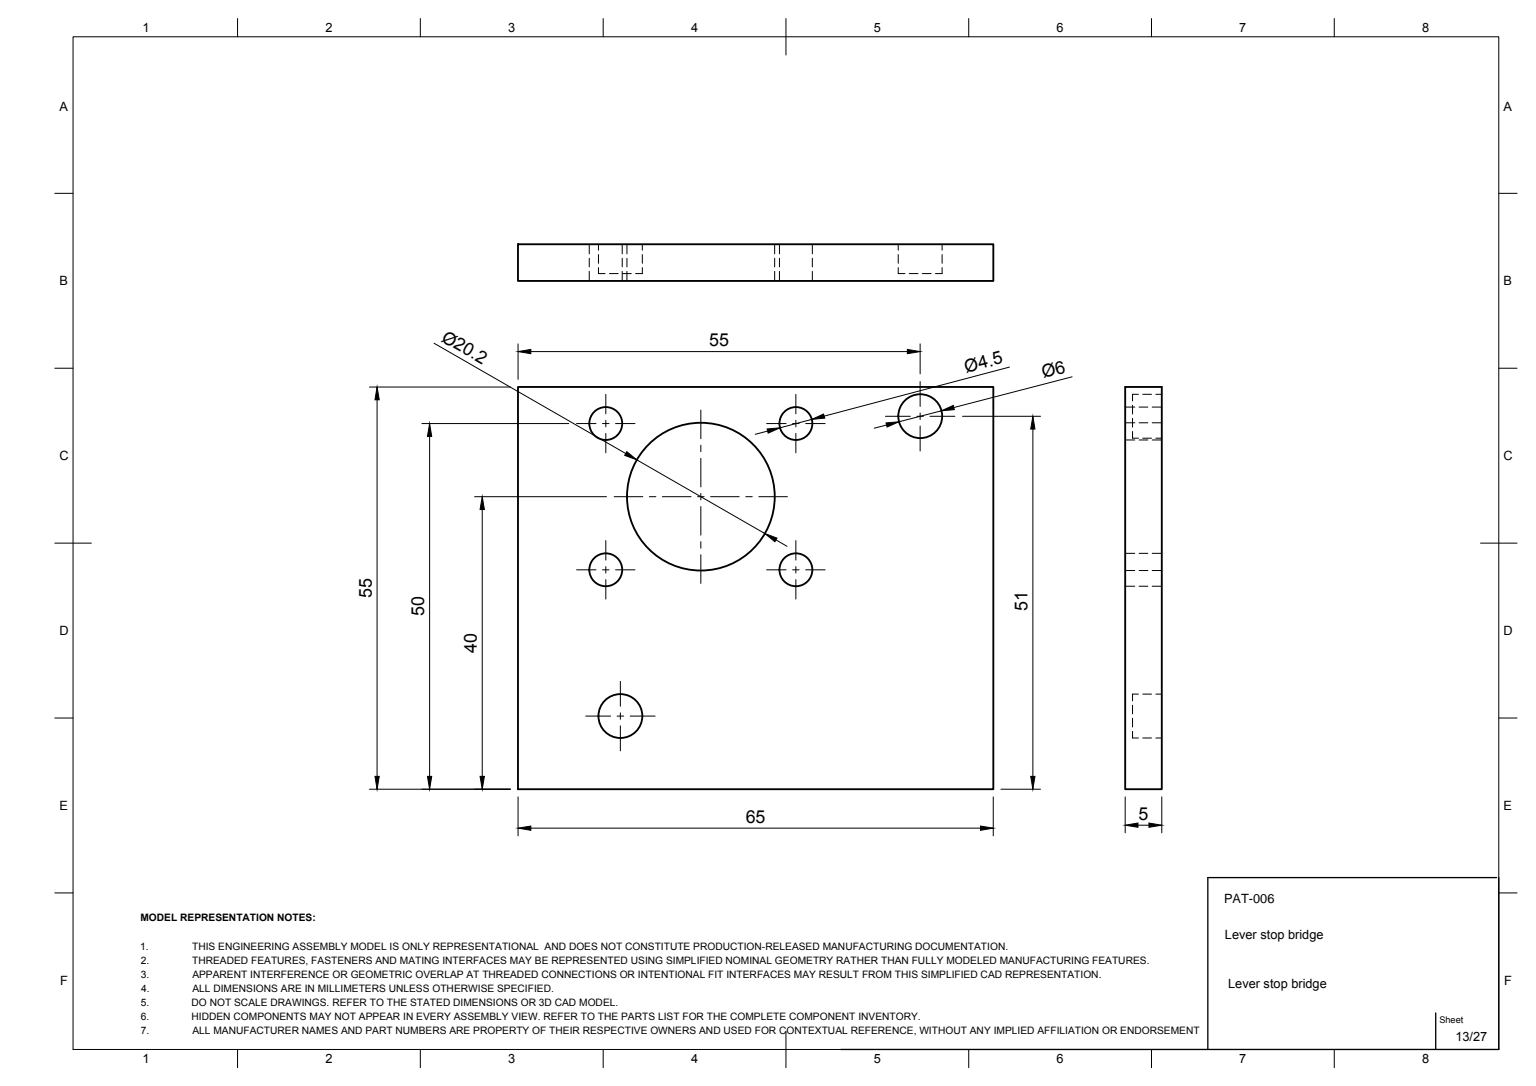
ISO-10303-21;
HEADER;
/* Generated by software containing ST-Developer
 * from STEP Tools, Inc. (www.steptools.com) 
 */

FILE_DESCRIPTION(
/* description */ ('Ball-type isolation valve (generic)'),
/* implementation_level */ '2;1');

FILE_NAME(
/* name */ 'Lever stop bridge.step',
/* time_stamp */ '2026-10-27T10:53:05-07:00',
/* author */ (''),
/* organization */ (''),
/* preprocessor_version */ 'ST-DEVELOPER v20.2',
/* originating_system */ 'Autodesk Translation Framework v15.17.0.0',
/* authorisation */ '');

FILE_SCHEMA (('AUTOMOTIVE_DESIGN { 1 0 10303 214 3 1 1 }'));
ENDSEC;

DATA;
#10=MECHANICAL_DESIGN_GEOMETRIC_PRESENTATION_REPRESENTATION('',(#285),#7425);
#233=SHAPE_REPRESENTATION_RELATIONSHIP('SRR','None',#7543,#259);
#259=ADVANCED_BREP_SHAPE_REPRESENTATION('',(#311),#7406);
#285=STYLED_ITEM('',(#7730),#311);
#311=MANIFOLD_SOLID_BREP('Body1',#4090);
#379=FACE_BOUND('',#971,.T.);
#380=FACE_BOUND('',#972,.T.);
#381=FACE_BOUND('',#973,.T.);
#382=FACE_BOUND('',#974,.T.);
#383=FACE_BOUND('',#975,.T.);
#384=FACE_BOUND('',#976,.T.);
#385=FACE_BOUND('',#977,.T.);
#386=FACE_BOUND('',#979,.T.);
#387=FACE_BOUND('',#980,.T.);
#388=FACE_BOUND('',#981,.T.);
#389=FACE_BOUND('',#982,.T.);
#390=FACE_BOUND('',#983,.T.);
#462=PLANE('',#4569);
#463=PLANE('',#4573);
#464=PLANE('',#4589);
#465=PLANE('',#4590);
#466=PLANE('',#4591);
#467=PLANE('',#4592);
#468=PLANE('',#4593);
#469=PLANE('',#4594);
#660=FACE_OUTER_BOUND('',#957,.T.);
#661=FACE_OUTER_BOUND('',#958,.T.);
#662=FACE_OUTER_BOUND('',#959,.T.);
#663=FACE_OUTER_BOUND('',#960,.T.);
#664=FACE_OUTER_BOUND('',#961,.T.);
#665=FACE_OUTER_BOUND('',#962,.T.);
#666=FACE_OUTER_BOUND('',#963,.T.);
#667=FACE_OUTER_BOUND('',#964,.T.);
#668=FACE_OUTER_BOUND('',#965,.T.);
#669=FACE_OUTER_BOUND('',#966,.T.);
#670=FACE_OUTER_BOUND('',#967,.T.);
#671=FACE_OUTER_BOUND('',#968,.T.);
#672=FACE_OUTER_BOUND('',#969,.T.);
#673=FACE_OUTER_BOUND('',#970,.T.);
#674=FACE_OUTER_BOUND('',#978,.T.);
#957=EDGE_LOOP('',(#3111,#3112,#3113,#3114));
#958=EDGE_LOOP('',(#3115));
#959=EDGE_LOOP('',(#3116,#3117,#3118,#3119));
#960=EDGE_LOOP('',(#3120));
#961=EDGE_LOOP('',(#3121,#3122,#3123,#3124));
#962=EDGE_LOOP('',(#3125,#3126,#3127,#3128));
#963=EDGE_LOOP('',(#3129,#3130,#3131,#3132));
#964=EDGE_LOOP('',(#3133,#3134,#3135,#3136));
#965=EDGE_LOOP('',(#3137,#3138,#3139,#3140));
#966=EDGE_LOOP('',(#3141,#3142,#3143,#3144));
#967=EDGE_LOOP('',(#3145,#3146,#3147,#3148));
#968=EDGE_LOOP('',(#3149,#3150,#3151,#3152));
#969=EDGE_LOOP('',(#3153,#3154,#3155,#3156));
#970=EDGE_LOOP('',(#3157,#3158,#3159,#3160));
#971=EDGE_LOOP('',(#3161));
#972=EDGE_LOOP('',(#3162));
#973=EDGE_LOOP('',(#3163));
#974=EDGE_LOOP('',(#3164));
#975=EDGE_LOOP('',(#3165));
#976=EDGE_LOOP('',(#3166));
#977=EDGE_LOOP('',(#3167));
#978=EDGE_LOOP('',(#3168,#3169,#3170,#3171));
#979=EDGE_LOOP('',(#3172));
#980=EDGE_LOOP('',(#3173));
#981=EDGE_LOOP('',(#3174));
#982=EDGE_LOOP('',(#3175));
#983=EDGE_LOOP('',(#3176));
#1257=LINE('',#6577,#1565);
#1258=LINE('',#6584,#1566);
#1259=LINE('',#6591,#1567);
#1260=LINE('',#6597,#1568);
#1261=LINE('',#6603,#1569);
#1262=LINE('',#6609,#1570);
#1263=LINE('',#6615,#1571);
#1264=LINE('',#6620,#1572);
#1265=LINE('',#6622,#1573);
#1266=LINE('',#6624,#1574);
#1267=LINE('',#6625,#1575);
#1268=LINE('',#6628,#1576);
#1269=LINE('',#6630,#1577);
#1270=LINE('',#6631,#1578);
#1271=LINE('',#6634,#1579);
#1272=LINE('',#6636,#1580);
#1273=LINE('',#6637,#1581);
#1274=LINE('',#6639,#1582);
#1275=LINE('',#6640,#1583);
#1565=VECTOR('',#5328,0.3);
#1566=VECTOR('',#5337,0.3);
#1567=VECTOR('',#5346,0.225);
#1568=VECTOR('',#5353,0.225);
#1569=VECTOR('',#5360,0.225);
#1570=VECTOR('',#5367,0.225);
#1571=VECTOR('',#5374,1.01);
#1572=VECTOR('',#5379,1.);
#1573=VECTOR('',#5380,1.);
#1574=VECTOR('',#5381,1.);
#1575=VECTOR('',#5382,1.);
#1576=VECTOR('',#5385,1.);
#1577=VECTOR('',#5386,1.);
#1578=VECTOR('',#5387,1.);
#1579=VECTOR('',#5390,1.);
#1580=VECTOR('',#5391,1.);
#1581=VECTOR('',#5392,1.);
#1582=VECTOR('',#5395,1.);
#1583=VECTOR('',#5396,1.);
#1857=CIRCLE('',#4567,0.3);
#1858=CIRCLE('',#4568,0.3);
#1859=CIRCLE('',#4571,0.3);
#1860=CIRCLE('',#4572,0.3);
#1861=CIRCLE('',#4575,0.225);
#1862=CIRCLE('',#4576,0.225);
#1863=CIRCLE('',#4578,0.225);
#1864=CIRCLE('',#4579,0.225);
#1865=CIRCLE('',#4581,0.225);
#1866=CIRCLE('',#4582,0.225);
#1867=CIRCLE('',#4584,0.225);
#1868=CIRCLE('',#4585,0.225);
#1869=CIRCLE('',#4587,1.01);
#1870=CIRCLE('',#4588,1.01);
#2069=VERTEX_POINT('',#6574);
#2070=VERTEX_POINT('',#6576);
#2071=VERTEX_POINT('',#6581);
#2072=VERTEX_POINT('',#6583);
#2073=VERTEX_POINT('',#6588);
#2074=VERTEX_POINT('',#6590);
#2075=VERTEX_POINT('',#6594);
#2076=VERTEX_POINT('',#6596);
#2077=VERTEX_POINT('',#6600);
#2078=VERTEX_POINT('',#6602);
#2079=VERTEX_POINT('',#6606);
#2080=VERTEX_POINT('',#6608);
#2081=VERTEX_POINT('',#6612);
#2082=VERTEX_POINT('',#6614);
#2083=VERTEX_POINT('',#6618);
#2084=VERTEX_POINT('',#6619);
#2085=VERTEX_POINT('',#6621);
#2086=VERTEX_POINT('',#6623);
#2087=VERTEX_POINT('',#6627);
#2088=VERTEX_POINT('',#6629);
#2089=VERTEX_POINT('',#6633);
#2090=VERTEX_POINT('',#6635);
#2448=EDGE_CURVE('',#2069,#2069,#1857,.T.);
#2449=EDGE_CURVE('',#2069,#2070,#1257,.T.);
#2450=EDGE_CURVE('',#2070,#2070,#1858,.T.);
#2451=EDGE_CURVE('',#2071,#2071,#1859,.T.);
#2452=EDGE_CURVE('',#2071,#2072,#1258,.T.);
#2453=EDGE_CURVE('',#2072,#2072,#1860,.T.);
#2454=EDGE_CURVE('',#2073,#2073,#1861,.T.);
#2455=EDGE_CURVE('',#2073,#2074,#1259,.T.);
#2456=EDGE_CURVE('',#2074,#2074,#1862,.T.);
#2457=EDGE_CURVE('',#2075,#2075,#1863,.T.);
#2458=EDGE_CURVE('',#2075,#2076,#1260,.T.);
#2459=EDGE_CURVE('',#2076,#2076,#1864,.T.);
#2460=EDGE_CURVE('',#2077,#2077,#1865,.T.);
#2461=EDGE_CURVE('',#2077,#2078,#1261,.T.);
#2462=EDGE_CURVE('',#2078,#2078,#1866,.T.);
#2463=EDGE_CURVE('',#2079,#2079,#1867,.T.);
#2464=EDGE_CURVE('',#2079,#2080,#1262,.T.);
#2465=EDGE_CURVE('',#2080,#2080,#1868,.T.);
#2466=EDGE_CURVE('',#2081,#2081,#1869,.T.);
#2467=EDGE_CURVE('',#2081,#2082,#1263,.T.);
#2468=EDGE_CURVE('',#2082,#2082,#1870,.T.);
#2469=EDGE_CURVE('',#2083,#2084,#1264,.T.);
#2470=EDGE_CURVE('',#2084,#2085,#1265,.T.);
#2471=EDGE_CURVE('',#2086,#2085,#1266,.T.);
#2472=EDGE_CURVE('',#2083,#2086,#1267,.T.);
#2473=EDGE_CURVE('',#2087,#2083,#1268,.T.);
#2474=EDGE_CURVE('',#2088,#2086,#1269,.T.);
#2475=EDGE_CURVE('',#2087,#2088,#1270,.T.);
#2476=EDGE_CURVE('',#2089,#2087,#1271,.T.);
#2477=EDGE_CURVE('',#2090,#2088,#1272,.T.);
#2478=EDGE_CURVE('',#2089,#2090,#1273,.T.);
#2479=EDGE_CURVE('',#2084,#2089,#1274,.T.);
#2480=EDGE_CURVE('',#2085,#2090,#1275,.T.);
#3111=ORIENTED_EDGE('',*,*,#2448,.F.);
#3112=ORIENTED_EDGE('',*,*,#2449,.T.);
#3113=ORIENTED_EDGE('',*,*,#2450,.F.);
#3114=ORIENTED_EDGE('',*,*,#2449,.F.);
#3115=ORIENTED_EDGE('',*,*,#2448,.T.);
#3116=ORIENTED_EDGE('',*,*,#2451,.F.);
#3117=ORIENTED_EDGE('',*,*,#2452,.T.);
#3118=ORIENTED_EDGE('',*,*,#2453,.F.);
#3119=ORIENTED_EDGE('',*,*,#2452,.F.);
#3120=ORIENTED_EDGE('',*,*,#2451,.T.);
#3121=ORIENTED_EDGE('',*,*,#2454,.F.);
#3122=ORIENTED_EDGE('',*,*,#2455,.T.);
#3123=ORIENTED_EDGE('',*,*,#2456,.F.);
#3124=ORIENTED_EDGE('',*,*,#2455,.F.);
#3125=ORIENTED_EDGE('',*,*,#2457,.F.);
#3126=ORIENTED_EDGE('',*,*,#2458,.T.);
#3127=ORIENTED_EDGE('',*,*,#2459,.F.);
#3128=ORIENTED_EDGE('',*,*,#2458,.F.);
#3129=ORIENTED_EDGE('',*,*,#2460,.F.);
#3130=ORIENTED_EDGE('',*,*,#2461,.T.);
#3131=ORIENTED_EDGE('',*,*,#2462,.F.);
#3132=ORIENTED_EDGE('',*,*,#2461,.F.);
#3133=ORIENTED_EDGE('',*,*,#2463,.F.);
#3134=ORIENTED_EDGE('',*,*,#2464,.T.);
#3135=ORIENTED_EDGE('',*,*,#2465,.F.);
#3136=ORIENTED_EDGE('',*,*,#2464,.F.);
#3137=ORIENTED_EDGE('',*,*,#2466,.F.);
#3138=ORIENTED_EDGE('',*,*,#2467,.T.);
#3139=ORIENTED_EDGE('',*,*,#2468,.F.);
#3140=ORIENTED_EDGE('',*,*,#2467,.F.);
#3141=ORIENTED_EDGE('',*,*,#2469,.T.);
#3142=ORIENTED_EDGE('',*,*,#2470,.T.);
#3143=ORIENTED_EDGE('',*,*,#2471,.F.);
#3144=ORIENTED_EDGE('',*,*,#2472,.F.);
#3145=ORIENTED_EDGE('',*,*,#2473,.T.);
#3146=ORIENTED_EDGE('',*,*,#2472,.T.);
#3147=ORIENTED_EDGE('',*,*,#2474,.F.);
#3148=ORIENTED_EDGE('',*,*,#2475,.F.);
#3149=ORIENTED_EDGE('',*,*,#2476,.T.);
#3150=ORIENTED_EDGE('',*,*,#2475,.T.);
#3151=ORIENTED_EDGE('',*,*,#2477,.F.);
#3152=ORIENTED_EDGE('',*,*,#2478,.F.);
#3153=ORIENTED_EDGE('',*,*,#2479,.T.);
#3154=ORIENTED_EDGE('',*,*,#2478,.T.);
#3155=ORIENTED_EDGE('',*,*,#2480,.F.);
#3156=ORIENTED_EDGE('',*,*,#2470,.F.);
#3157=ORIENTED_EDGE('',*,*,#2480,.T.);
#3158=ORIENTED_EDGE('',*,*,#2477,.T.);
#3159=ORIENTED_EDGE('',*,*,#2474,.T.);
#3160=ORIENTED_EDGE('',*,*,#2471,.T.);
#3161=ORIENTED_EDGE('',*,*,#2450,.T.);
#3162=ORIENTED_EDGE('',*,*,#2453,.T.);
#3163=ORIENTED_EDGE('',*,*,#2468,.T.);
#3164=ORIENTED_EDGE('',*,*,#2465,.T.);
#3165=ORIENTED_EDGE('',*,*,#2462,.T.);
#3166=ORIENTED_EDGE('',*,*,#2459,.T.);
#3167=ORIENTED_EDGE('',*,*,#2456,.T.);
#3168=ORIENTED_EDGE('',*,*,#2479,.F.);
#3169=ORIENTED_EDGE('',*,*,#2469,.F.);
#3170=ORIENTED_EDGE('',*,*,#2473,.F.);
#3171=ORIENTED_EDGE('',*,*,#2476,.F.);
#3172=ORIENTED_EDGE('',*,*,#2466,.T.);
#3173=ORIENTED_EDGE('',*,*,#2463,.T.);
#3174=ORIENTED_EDGE('',*,*,#2460,.T.);
#3175=ORIENTED_EDGE('',*,*,#2457,.T.);
#3176=ORIENTED_EDGE('',*,*,#2454,.T.);
#3798=CYLINDRICAL_SURFACE('',#4566,0.3);
#3799=CYLINDRICAL_SURFACE('',#4570,0.3);
#3800=CYLINDRICAL_SURFACE('',#4574,0.225);
#3801=CYLINDRICAL_SURFACE('',#4577,0.225);
#3802=CYLINDRICAL_SURFACE('',#4580,0.225);
#3803=CYLINDRICAL_SURFACE('',#4583,0.225);
#3804=CYLINDRICAL_SURFACE('',#4586,1.01);
#3914=ADVANCED_FACE('',(#660),#3798,.F.);
#3915=ADVANCED_FACE('',(#661),#462,.T.);
#3916=ADVANCED_FACE('',(#662),#3799,.F.);
#3917=ADVANCED_FACE('',(#663),#463,.T.);
#3918=ADVANCED_FACE('',(#664),#3800,.F.);
#3919=ADVANCED_FACE('',(#665),#3801,.F.);
#3920=ADVANCED_FACE('',(#666),#3802,.F.);
#3921=ADVANCED_FACE('',(#667),#3803,.F.);
#3922=ADVANCED_FACE('',(#668),#3804,.F.);
#3923=ADVANCED_FACE('',(#669),#464,.T.);
#3924=ADVANCED_FACE('',(#670),#465,.T.);
#3925=ADVANCED_FACE('',(#671),#466,.T.);
#3926=ADVANCED_FACE('',(#672),#467,.T.);
#3927=ADVANCED_FACE('',(#673,#379,#380,#381,#382,#383,#384,#385),#468,.T.);
#3928=ADVANCED_FACE('',(#674,#386,#387,#388,#389,#390),#469,.F.);
#4090=CLOSED_SHELL('',(#3914,#3915,#3916,#3917,#3918,#3919,#3920,#3921,
#3922,#3923,#3924,#3925,#3926,#3927,#3928));
#4565=AXIS2_PLACEMENT_3D('',#6572,#5322,#5323);
#4566=AXIS2_PLACEMENT_3D('',#6573,#5324,#5325);
#4567=AXIS2_PLACEMENT_3D('',#6575,#5326,#5327);
#4568=AXIS2_PLACEMENT_3D('',#6578,#5329,#5330);
#4569=AXIS2_PLACEMENT_3D('',#6579,#5331,#5332);
#4570=AXIS2_PLACEMENT_3D('',#6580,#5333,#5334);
#4571=AXIS2_PLACEMENT_3D('',#6582,#5335,#5336);
#4572=AXIS2_PLACEMENT_3D('',#6585,#5338,#5339);
#4573=AXIS2_PLACEMENT_3D('',#6586,#5340,#5341);
#4574=AXIS2_PLACEMENT_3D('',#6587,#5342,#5343);
#4575=AXIS2_PLACEMENT_3D('',#6589,#5344,#5345);
#4576=AXIS2_PLACEMENT_3D('',#6592,#5347,#5348);
#4577=AXIS2_PLACEMENT_3D('',#6593,#5349,#5350);
#4578=AXIS2_PLACEMENT_3D('',#6595,#5351,#5352);
#4579=AXIS2_PLACEMENT_3D('',#6598,#5354,#5355);
#4580=AXIS2_PLACEMENT_3D('',#6599,#5356,#5357);
#4581=AXIS2_PLACEMENT_3D('',#6601,#5358,#5359);
#4582=AXIS2_PLACEMENT_3D('',#6604,#5361,#5362);
#4583=AXIS2_PLACEMENT_3D('',#6605,#5363,#5364);
#4584=AXIS2_PLACEMENT_3D('',#6607,#5365,#5366);
#4585=AXIS2_PLACEMENT_3D('',#6610,#5368,#5369);
#4586=AXIS2_PLACEMENT_3D('',#6611,#5370,#5371);
#4587=AXIS2_PLACEMENT_3D('',#6613,#5372,#5373);
#4588=AXIS2_PLACEMENT_3D('',#6616,#5375,#5376);
#4589=AXIS2_PLACEMENT_3D('',#6617,#5377,#5378);
#4590=AXIS2_PLACEMENT_3D('',#6626,#5383,#5384);
#4591=AXIS2_PLACEMENT_3D('',#6632,#5388,#5389);
#4592=AXIS2_PLACEMENT_3D('',#6638,#5393,#5394);
#4593=AXIS2_PLACEMENT_3D('',#6641,#5397,#5398);
#4594=AXIS2_PLACEMENT_3D('',#6642,#5399,#5400);
#5322=DIRECTION('axis',(0.,0.,1.));
#5323=DIRECTION('refdir',(1.,0.,0.));
#5324=DIRECTION('center_axis',(0.,0.,1.));
#5325=DIRECTION('ref_axis',(1.,0.,0.));
#5326=DIRECTION('center_axis',(0.,0.,1.));
#5327=DIRECTION('ref_axis',(1.,0.,0.));
#5328=DIRECTION('',(0.,0.,1.));
#5329=DIRECTION('center_axis',(0.,0.,-1.));
#5330=DIRECTION('ref_axis',(1.,0.,0.));
#5331=DIRECTION('center_axis',(0.,0.,1.));
#5332=DIRECTION('ref_axis',(1.,0.,0.));
#5333=DIRECTION('center_axis',(0.,0.,1.));
#5334=DIRECTION('ref_axis',(1.,0.,0.));
#5335=DIRECTION('center_axis',(0.,0.,1.));
#5336=DIRECTION('ref_axis',(1.,0.,0.));
#5337=DIRECTION('',(0.,0.,1.));
#5338=DIRECTION('center_axis',(0.,0.,-1.));
#5339=DIRECTION('ref_axis',(1.,0.,0.));
#5340=DIRECTION('center_axis',(0.,0.,1.));
#5341=DIRECTION('ref_axis',(1.,0.,0.));
#5342=DIRECTION('center_axis',(0.,0.,1.));
#5343=DIRECTION('ref_axis',(1.,0.,0.));
#5344=DIRECTION('center_axis',(0.,0.,1.));
#5345=DIRECTION('ref_axis',(1.,0.,0.));
#5346=DIRECTION('',(0.,0.,1.));
#5347=DIRECTION('center_axis',(0.,0.,-1.));
#5348=DIRECTION('ref_axis',(1.,0.,0.));
#5349=DIRECTION('center_axis',(0.,0.,1.));
#5350=DIRECTION('ref_axis',(1.,0.,0.));
#5351=DIRECTION('center_axis',(0.,0.,1.));
#5352=DIRECTION('ref_axis',(1.,0.,0.));
#5353=DIRECTION('',(0.,0.,1.));
#5354=DIRECTION('center_axis',(0.,0.,-1.));
#5355=DIRECTION('ref_axis',(1.,0.,0.));
#5356=DIRECTION('center_axis',(0.,0.,1.));
#5357=DIRECTION('ref_axis',(1.,0.,0.));
#5358=DIRECTION('center_axis',(0.,0.,1.));
#5359=DIRECTION('ref_axis',(1.,0.,0.));
#5360=DIRECTION('',(0.,0.,1.));
#5361=DIRECTION('center_axis',(0.,0.,-1.));
#5362=DIRECTION('ref_axis',(1.,0.,0.));
#5363=DIRECTION('center_axis',(0.,0.,1.));
#5364=DIRECTION('ref_axis',(1.,0.,0.));
#5365=DIRECTION('center_axis',(0.,0.,1.));
#5366=DIRECTION('ref_axis',(1.,0.,0.));
#5367=DIRECTION('',(0.,0.,1.));
#5368=DIRECTION('center_axis',(0.,0.,-1.));
#5369=DIRECTION('ref_axis',(1.,0.,0.));
#5370=DIRECTION('center_axis',(0.,0.,1.));
#5371=DIRECTION('ref_axis',(1.,0.,0.));
#5372=DIRECTION('center_axis',(0.,0.,1.));
#5373=DIRECTION('ref_axis',(1.,0.,0.));
#5374=DIRECTION('',(0.,0.,1.));
#5375=DIRECTION('center_axis',(0.,0.,-1.));
#5376=DIRECTION('ref_axis',(1.,0.,0.));
#5377=DIRECTION('center_axis',(0.,1.,0.));
#5378=DIRECTION('ref_axis',(-1.,0.,0.));
#5379=DIRECTION('',(-1.,0.,0.));
#5380=DIRECTION('',(0.,0.,1.));
#5381=DIRECTION('',(-1.,0.,0.));
#5382=DIRECTION('',(0.,0.,1.));
#5383=DIRECTION('center_axis',(1.,0.,0.));
#5384=DIRECTION('ref_axis',(0.,1.,0.));
#5385=DIRECTION('',(0.,1.,0.));
#5386=DIRECTION('',(0.,1.,0.));
#5387=DIRECTION('',(0.,0.,1.));
#5388=DIRECTION('center_axis',(0.,-1.,0.));
#5389=DIRECTION('ref_axis',(1.,0.,0.));
#5390=DIRECTION('',(1.,0.,0.));
#5391=DIRECTION('',(1.,0.,0.));
#5392=DIRECTION('',(0.,0.,1.));
#5393=DIRECTION('center_axis',(-1.,0.,0.));
#5394=DIRECTION('ref_axis',(0.,-1.,0.));
#5395=DIRECTION('',(0.,-1.,0.));
#5396=DIRECTION('',(0.,-1.,0.));
#5397=DIRECTION('center_axis',(0.,0.,1.));
#5398=DIRECTION('ref_axis',(1.,0.,0.));
#5399=DIRECTION('center_axis',(0.,0.,1.));
#5400=DIRECTION('ref_axis',(1.,0.,0.));
#6572=CARTESIAN_POINT('',(0.,0.,0.));
#6573=CARTESIAN_POINT('Origin',(-1.1,-3.,8.1));
#6574=CARTESIAN_POINT('',(-1.4,-3.,8.1));
#6575=CARTESIAN_POINT('Origin',(-1.1,-3.,8.1));
#6576=CARTESIAN_POINT('',(-1.4,-3.,8.5));
#6577=CARTESIAN_POINT('',(-1.4,-3.,8.1));
#6578=CARTESIAN_POINT('Origin',(-1.1,-3.,8.5));
#6579=CARTESIAN_POINT('Origin',(-1.1,-3.,8.1));
#6580=CARTESIAN_POINT('Origin',(3.,1.1,8.1));
#6581=CARTESIAN_POINT('',(2.7,1.1,8.1));
#6582=CARTESIAN_POINT('Origin',(3.,1.1,8.1));
#6583=CARTESIAN_POINT('',(2.7,1.1,8.5));
#6584=CARTESIAN_POINT('',(2.7,1.1,8.1));
#6585=CARTESIAN_POINT('Origin',(3.,1.1,8.5));
#6586=CARTESIAN_POINT('Origin',(3.,1.1,8.1));
#6587=CARTESIAN_POINT('Origin',(1.3,-1.,7.9));
#6588=CARTESIAN_POINT('',(1.075,-1.,8.));
#6589=CARTESIAN_POINT('Origin',(1.3,-1.,8.));
#6590=CARTESIAN_POINT('',(1.075,-1.,8.5));
#6591=CARTESIAN_POINT('',(1.075,-1.,7.9));
#6592=CARTESIAN_POINT('Origin',(1.3,-1.,8.5));
#6593=CARTESIAN_POINT('Origin',(-1.3,1.,7.9));
#6594=CARTESIAN_POINT('',(-1.525,1.,8.));
#6595=CARTESIAN_POINT('Origin',(-1.3,1.,8.));
#6596=CARTESIAN_POINT('',(-1.525,1.,8.5));
#6597=CARTESIAN_POINT('',(-1.525,1.,7.9));
#6598=CARTESIAN_POINT('Origin',(-1.3,1.,8.5));
#6599=CARTESIAN_POINT('Origin',(-1.3,-1.,7.9));
#6600=CARTESIAN_POINT('',(-1.525,-1.,8.));
#6601=CARTESIAN_POINT('Origin',(-1.3,-1.,8.));
#6602=CARTESIAN_POINT('',(-1.525,-1.,8.5));
#6603=CARTESIAN_POINT('',(-1.525,-1.,7.9));
#6604=CARTESIAN_POINT('Origin',(-1.3,-1.,8.5));
#6605=CARTESIAN_POINT('Origin',(1.3,1.,7.9));
#6606=CARTESIAN_POINT('',(1.075,1.,8.));
#6607=CARTESIAN_POINT('Origin',(1.3,1.,8.));
#6608=CARTESIAN_POINT('',(1.075,1.,8.5));
#6609=CARTESIAN_POINT('',(1.075,1.,7.9));
#6610=CARTESIAN_POINT('Origin',(1.3,1.,8.5));
#6611=CARTESIAN_POINT('Origin',(0.,0.,7.9));
#6612=CARTESIAN_POINT('',(-1.01,-1.23689326713883E-16,8.));
#6613=CARTESIAN_POINT('Origin',(0.,0.,8.));
#6614=CARTESIAN_POINT('',(-1.01,1.23689326713883E-16,8.5));
#6615=CARTESIAN_POINT('',(-1.01,-1.23689326713883E-16,7.9));
#6616=CARTESIAN_POINT('Origin',(0.,0.,8.5));
#6617=CARTESIAN_POINT('Origin',(4.,1.5,8.));
#6618=CARTESIAN_POINT('',(4.,1.5,8.));
#6619=CARTESIAN_POINT('',(-2.5,1.5,8.));
#6620=CARTESIAN_POINT('',(4.,1.5,8.));
#6621=CARTESIAN_POINT('',(-2.5,1.5,8.5));
#6622=CARTESIAN_POINT('',(-2.5,1.5,8.));
#6623=CARTESIAN_POINT('',(4.,1.5,8.5));
#6624=CARTESIAN_POINT('',(4.,1.5,8.5));
#6625=CARTESIAN_POINT('',(4.,1.5,8.));
#6626=CARTESIAN_POINT('Origin',(4.,-4.,8.));
#6627=CARTESIAN_POINT('',(4.,-4.,8.));
#6628=CARTESIAN_POINT('',(4.,-4.,8.));
#6629=CARTESIAN_POINT('',(4.,-4.,8.5));
#6630=CARTESIAN_POINT('',(4.,-4.,8.5));
#6631=CARTESIAN_POINT('',(4.,-4.,8.));
#6632=CARTESIAN_POINT('Origin',(-2.5,-4.,8.));
#6633=CARTESIAN_POINT('',(-2.5,-4.,8.));
#6634=CARTESIAN_POINT('',(-2.5,-4.,8.));
#6635=CARTESIAN_POINT('',(-2.5,-4.,8.5));
#6636=CARTESIAN_POINT('',(-2.5,-4.,8.5));
#6637=CARTESIAN_POINT('',(-2.5,-4.,8.));
#6638=CARTESIAN_POINT('Origin',(-2.5,1.5,8.));
#6639=CARTESIAN_POINT('',(-2.5,1.5,8.));
#6640=CARTESIAN_POINT('',(-2.5,1.5,8.5));
#6641=CARTESIAN_POINT('Origin',(0.75,-1.25,8.5));
#6642=CARTESIAN_POINT('Origin',(0.75,-1.25,8.));
#7376=UNCERTAINTY_MEASURE_WITH_UNIT(LENGTH_MEASURE(0.001),#7426,
'DISTANCE_ACCURACY_VALUE',
'Maximum model space distance between geometric entities at asserted c
onnectivities');
#7395=UNCERTAINTY_MEASURE_WITH_UNIT(LENGTH_MEASURE(0.001),#7426,
'DISTANCE_ACCURACY_VALUE',
'Maximum model space distance between geometric entities at asserted c
onnectivities');
#7406=(
GEOMETRIC_REPRESENTATION_CONTEXT(3)
GLOBAL_UNCERTAINTY_ASSIGNED_CONTEXT((#7376))
GLOBAL_UNIT_ASSIGNED_CONTEXT((#7426,#7428,#7429))
REPRESENTATION_CONTEXT('','3D')
);
#7425=(
GEOMETRIC_REPRESENTATION_CONTEXT(3)
GLOBAL_UNCERTAINTY_ASSIGNED_CONTEXT((#7395))
GLOBAL_UNIT_ASSIGNED_CONTEXT((#7426,#7428,#7429))
REPRESENTATION_CONTEXT('','3D')
);
#7426=(
LENGTH_UNIT()
NAMED_UNIT(*)
SI_UNIT(.CENTI.,.METRE.)
);
#7428=(
NAMED_UNIT(*)
PLANE_ANGLE_UNIT()
SI_UNIT($,.RADIAN.)
);
#7429=(
NAMED_UNIT(*)
SI_UNIT($,.STERADIAN.)
SOLID_ANGLE_UNIT()
);
#7440=SHAPE_DEFINITION_REPRESENTATION(#7469,#7543);
#7469=PRODUCT_DEFINITION_SHAPE('',$,#7573);
#7543=SHAPE_REPRESENTATION('',(#4565),#7406);
#7562=PRODUCT_DEFINITION_CONTEXT('part definition',#7651,'design');
#7573=PRODUCT_DEFINITION('Lever stop bridge','Lever stop bridge',#7602,
#7562);
#7602=PRODUCT_DEFINITION_FORMATION('',$,#7663);
#7651=APPLICATION_CONTEXT(
'Core Data for Automotive Mechanical Design Process');
#7652=PRODUCT_CONTEXT('part definition',#7651,'mechanical');
#7663=PRODUCT('Lever stop bridge','Lever stop bridge',
'Lever stop bridge',(#7652));
#7724=COLOUR_RGB('Light Blue',0.38,0.62,0.78);
#7725=FILL_AREA_STYLE_COLOUR('',#7724);
#7726=FILL_AREA_STYLE('',(#7725));
#7727=SURFACE_STYLE_FILL_AREA(#7726);
#7728=SURFACE_SIDE_STYLE('',(#7727));
#7729=SURFACE_STYLE_USAGE(.BOTH.,#7728);
#7730=PRESENTATION_STYLE_ASSIGNMENT((#7729));
ENDSEC;
END-ISO-10303-21;
